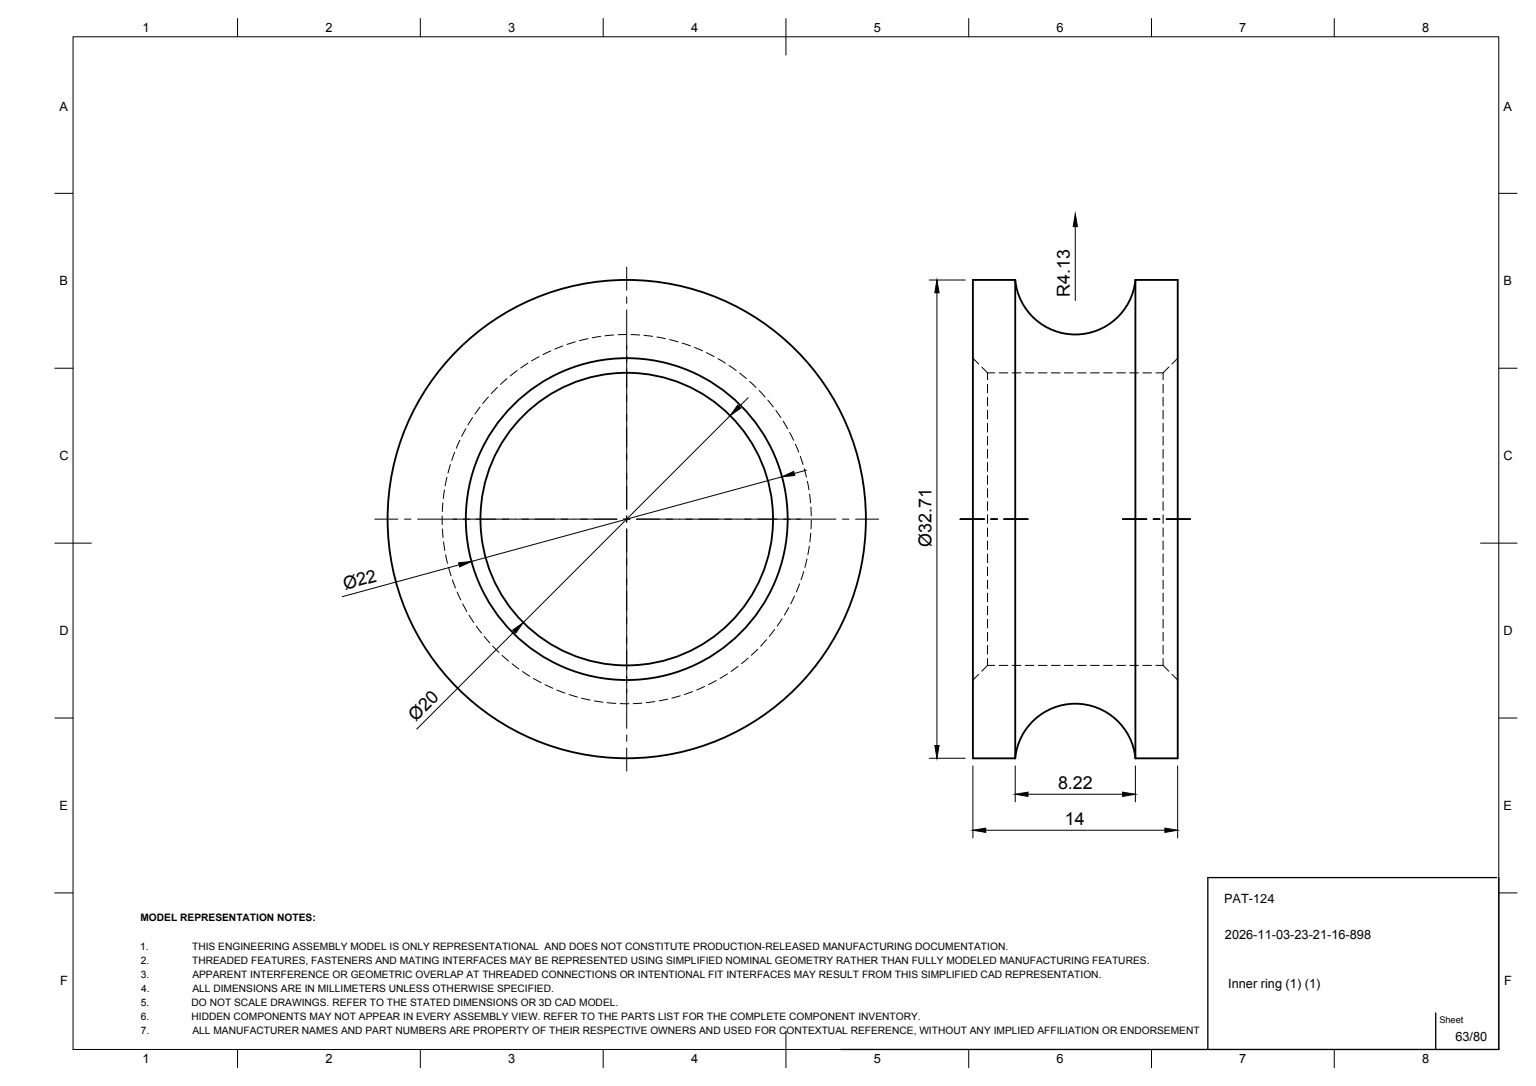
ISO-10303-21;
HEADER;
/* Generated by software containing ST-Developer
 * from STEP Tools, Inc. (www.steptools.com) 
 */

FILE_DESCRIPTION(
/* description */ ('XY cross-slide table'),
/* implementation_level */ '2;1');

FILE_NAME(
/* name */ 'Inner ring (1) (1).step',
/* time_stamp */ '2026-10-28T03:22:46-07:00',
/* author */ (''),
/* organization */ (''),
/* preprocessor_version */ 'ST-DEVELOPER v20.2',
/* originating_system */ 'Autodesk Translation Framework v15.17.0.0',
/* authorisation */ '');

FILE_SCHEMA (('AUTOMOTIVE_DESIGN { 1 0 10303 214 3 1 1 }'));
ENDSEC;

DATA;
#10=MECHANICAL_DESIGN_GEOMETRIC_PRESENTATION_REPRESENTATION('',(#1748),#62984);
#1471=CONICAL_SURFACE('',#25671,1.05,0.785398163397449);
#1472=CONICAL_SURFACE('',#25678,1.05,0.785398163397449);
#1502=TOROIDAL_SURFACE('',#25660,1.675,0.412776);
#1560=SHAPE_REPRESENTATION_RELATIONSHIP('SRR','None',#63417,#1643);
#1643=ADVANCED_BREP_SHAPE_REPRESENTATION('',(#1857),#62954);
#1748=STYLED_ITEM('',(#63912),#1857);
#1857=MANIFOLD_SOLID_BREP('Body1',#23046);
#2210=FACE_BOUND('',#5365,.T.);
#2211=FACE_BOUND('',#5368,.T.);
#2678=PLANE('',#25673);
#2679=PLANE('',#25676);
#3723=FACE_OUTER_BOUND('',#5360,.T.);
#3724=FACE_OUTER_BOUND('',#5361,.T.);
#3725=FACE_OUTER_BOUND('',#5362,.T.);
#3726=FACE_OUTER_BOUND('',#5363,.T.);
#3727=FACE_OUTER_BOUND('',#5364,.T.);
#3728=FACE_OUTER_BOUND('',#5366,.T.);
#3729=FACE_OUTER_BOUND('',#5367,.T.);
#3730=FACE_OUTER_BOUND('',#5369,.T.);
#5360=EDGE_LOOP('',(#18826,#18827,#18828,#18829,#18830,#18831));
#5361=EDGE_LOOP('',(#18832,#18833,#18834,#18835,#18836));
#5362=EDGE_LOOP('',(#18837,#18838,#18839,#18840));
#5363=EDGE_LOOP('',(#18841,#18842,#18843,#18844));
#5364=EDGE_LOOP('',(#18845));
#5365=EDGE_LOOP('',(#18846));
#5366=EDGE_LOOP('',(#18847,#18848,#18849,#18850,#18851));
#5367=EDGE_LOOP('',(#18852));
#5368=EDGE_LOOP('',(#18853));
#5369=EDGE_LOOP('',(#18854,#18855,#18856,#18857));
#6853=LINE('',#49072,#8340);
#6854=LINE('',#49078,#8341);
#6855=LINE('',#49082,#8342);
#6856=LINE('',#49088,#8343);
#6857=LINE('',#49093,#8344);
#8340=VECTOR('',#30742,1.63531);
#8341=VECTOR('',#30749,1.);
#8342=VECTOR('',#30754,1.05);
#8343=VECTOR('',#30763,1.63531);
#8344=VECTOR('',#30770,1.05);
#9536=CIRCLE('',#25661,1.63531);
#9537=CIRCLE('',#25662,1.63531);
#9538=CIRCLE('',#25663,0.412776);
#9539=CIRCLE('',#25664,1.63531);
#9540=CIRCLE('',#25665,1.63531);
#9541=CIRCLE('',#25667,1.63531);
#9542=CIRCLE('',#25669,1.);
#9543=CIRCLE('',#25670,1.);
#9544=CIRCLE('',#25672,1.1);
#9545=CIRCLE('',#25675,1.63531);
#9546=CIRCLE('',#25677,1.1);
#11095=VERTEX_POINT('',#49061);
#11096=VERTEX_POINT('',#49062);
#11097=VERTEX_POINT('',#49065);
#11098=VERTEX_POINT('',#49067);
#11099=VERTEX_POINT('',#49071);
#11100=VERTEX_POINT('',#49075);
#11101=VERTEX_POINT('',#49077);
#11102=VERTEX_POINT('',#49081);
#11103=VERTEX_POINT('',#49086);
#11104=VERTEX_POINT('',#49090);
#13797=EDGE_CURVE('',#11095,#11096,#9536,.T.);
#13798=EDGE_CURVE('',#11096,#11095,#9537,.T.);
#13799=EDGE_CURVE('',#11096,#11097,#9538,.T.);
#13800=EDGE_CURVE('',#11098,#11097,#9539,.T.);
#13801=EDGE_CURVE('',#11097,#11098,#9540,.T.);
#13802=EDGE_CURVE('',#11098,#11099,#6853,.T.);
#13803=EDGE_CURVE('',#11099,#11099,#9541,.T.);
#13804=EDGE_CURVE('',#11100,#11100,#9542,.T.);
#13805=EDGE_CURVE('',#11100,#11101,#6854,.T.);
#13806=EDGE_CURVE('',#11101,#11101,#9543,.T.);
#13807=EDGE_CURVE('',#11101,#11102,#6855,.T.);
#13808=EDGE_CURVE('',#11102,#11102,#9544,.T.);
#13809=EDGE_CURVE('',#11103,#11103,#9545,.T.);
#13810=EDGE_CURVE('',#11103,#11095,#6856,.T.);
#13811=EDGE_CURVE('',#11104,#11104,#9546,.T.);
#13812=EDGE_CURVE('',#11104,#11100,#6857,.T.);
#18826=ORIENTED_EDGE('',*,*,#13797,.F.);
#18827=ORIENTED_EDGE('',*,*,#13798,.F.);
#18828=ORIENTED_EDGE('',*,*,#13799,.T.);
#18829=ORIENTED_EDGE('',*,*,#13800,.F.);
#18830=ORIENTED_EDGE('',*,*,#13801,.F.);
#18831=ORIENTED_EDGE('',*,*,#13799,.F.);
#18832=ORIENTED_EDGE('',*,*,#13800,.T.);
#18833=ORIENTED_EDGE('',*,*,#13801,.T.);
#18834=ORIENTED_EDGE('',*,*,#13802,.T.);
#18835=ORIENTED_EDGE('',*,*,#13803,.T.);
#18836=ORIENTED_EDGE('',*,*,#13802,.F.);
#18837=ORIENTED_EDGE('',*,*,#13804,.T.);
#18838=ORIENTED_EDGE('',*,*,#13805,.T.);
#18839=ORIENTED_EDGE('',*,*,#13806,.F.);
#18840=ORIENTED_EDGE('',*,*,#13805,.F.);
#18841=ORIENTED_EDGE('',*,*,#13806,.T.);
#18842=ORIENTED_EDGE('',*,*,#13807,.T.);
#18843=ORIENTED_EDGE('',*,*,#13808,.F.);
#18844=ORIENTED_EDGE('',*,*,#13807,.F.);
#18845=ORIENTED_EDGE('',*,*,#13803,.F.);
#18846=ORIENTED_EDGE('',*,*,#13808,.T.);
#18847=ORIENTED_EDGE('',*,*,#13809,.F.);
#18848=ORIENTED_EDGE('',*,*,#13810,.T.);
#18849=ORIENTED_EDGE('',*,*,#13797,.T.);
#18850=ORIENTED_EDGE('',*,*,#13798,.T.);
#18851=ORIENTED_EDGE('',*,*,#13810,.F.);
#18852=ORIENTED_EDGE('',*,*,#13809,.T.);
#18853=ORIENTED_EDGE('',*,*,#13811,.F.);
#18854=ORIENTED_EDGE('',*,*,#13811,.T.);
#18855=ORIENTED_EDGE('',*,*,#13812,.T.);
#18856=ORIENTED_EDGE('',*,*,#13804,.F.);
#18857=ORIENTED_EDGE('',*,*,#13812,.F.);
#21428=CYLINDRICAL_SURFACE('',#25666,1.63531);
#21429=CYLINDRICAL_SURFACE('',#25668,1.);
#21430=CYLINDRICAL_SURFACE('',#25674,1.63531);
#22504=ADVANCED_FACE('',(#3723),#1502,.F.);
#22505=ADVANCED_FACE('',(#3724),#21428,.T.);
#22506=ADVANCED_FACE('',(#3725),#21429,.F.);
#22507=ADVANCED_FACE('',(#3726),#1471,.F.);
#22508=ADVANCED_FACE('',(#3727,#2210),#2678,.T.);
#22509=ADVANCED_FACE('',(#3728),#21430,.T.);
#22510=ADVANCED_FACE('',(#3729,#2211),#2679,.T.);
#22511=ADVANCED_FACE('',(#3730),#1472,.F.);
#23046=CLOSED_SHELL('',(#22504,#22505,#22506,#22507,#22508,#22509,#22510,
#22511));
#25659=AXIS2_PLACEMENT_3D('',#49059,#30726,#30727);
#25660=AXIS2_PLACEMENT_3D('',#49060,#30728,#30729);
#25661=AXIS2_PLACEMENT_3D('',#49063,#30730,#30731);
#25662=AXIS2_PLACEMENT_3D('',#49064,#30732,#30733);
#25663=AXIS2_PLACEMENT_3D('',#49066,#30734,#30735);
#25664=AXIS2_PLACEMENT_3D('',#49068,#30736,#30737);
#25665=AXIS2_PLACEMENT_3D('',#49069,#30738,#30739);
#25666=AXIS2_PLACEMENT_3D('',#49070,#30740,#30741);
#25667=AXIS2_PLACEMENT_3D('',#49073,#30743,#30744);
#25668=AXIS2_PLACEMENT_3D('',#49074,#30745,#30746);
#25669=AXIS2_PLACEMENT_3D('',#49076,#30747,#30748);
#25670=AXIS2_PLACEMENT_3D('',#49079,#30750,#30751);
#25671=AXIS2_PLACEMENT_3D('',#49080,#30752,#30753);
#25672=AXIS2_PLACEMENT_3D('',#49083,#30755,#30756);
#25673=AXIS2_PLACEMENT_3D('',#49084,#30757,#30758);
#25674=AXIS2_PLACEMENT_3D('',#49085,#30759,#30760);
#25675=AXIS2_PLACEMENT_3D('',#49087,#30761,#30762);
#25676=AXIS2_PLACEMENT_3D('',#49089,#30764,#30765);
#25677=AXIS2_PLACEMENT_3D('',#49091,#30766,#30767);
#25678=AXIS2_PLACEMENT_3D('',#49092,#30768,#30769);
#30726=DIRECTION('axis',(0.,0.,1.));
#30727=DIRECTION('refdir',(1.,0.,0.));
#30728=DIRECTION('center_axis',(0.,-1.,0.));
#30729=DIRECTION('ref_axis',(0.,0.,-1.));
#30730=DIRECTION('center_axis',(0.,-1.,0.));
#30731=DIRECTION('ref_axis',(1.,0.,0.));
#30732=DIRECTION('center_axis',(0.,-1.,0.));
#30733=DIRECTION('ref_axis',(1.,0.,0.));
#30734=DIRECTION('center_axis',(1.,0.,1.22464679914735E-16));
#30735=DIRECTION('ref_axis',(-1.22464679914735E-16,0.,1.));
#30736=DIRECTION('center_axis',(0.,1.,0.));
#30737=DIRECTION('ref_axis',(1.,0.,0.));
#30738=DIRECTION('center_axis',(0.,1.,0.));
#30739=DIRECTION('ref_axis',(1.,0.,0.));
#30740=DIRECTION('center_axis',(0.,-1.,0.));
#30741=DIRECTION('ref_axis',(1.,0.,0.));
#30742=DIRECTION('',(0.,1.,0.));
#30743=DIRECTION('center_axis',(0.,-1.,0.));
#30744=DIRECTION('ref_axis',(1.,0.,0.));
#30745=DIRECTION('center_axis',(0.,-1.,0.));
#30746=DIRECTION('ref_axis',(1.,0.,0.));
#30747=DIRECTION('center_axis',(0.,-1.,0.));
#30748=DIRECTION('ref_axis',(1.,0.,0.));
#30749=DIRECTION('',(0.,1.,0.));
#30750=DIRECTION('center_axis',(0.,-1.,0.));
#30751=DIRECTION('ref_axis',(1.,0.,0.));
#30752=DIRECTION('center_axis',(0.,1.,0.));
#30753=DIRECTION('ref_axis',(1.,0.,0.));
#30754=DIRECTION('',(-0.707106781186548,0.707106781186547,-8.65956056235494E-17));
#30755=DIRECTION('center_axis',(0.,-1.,0.));
#30756=DIRECTION('ref_axis',(1.,0.,0.));
#30757=DIRECTION('center_axis',(0.,1.,0.));
#30758=DIRECTION('ref_axis',(0.,0.,1.));
#30759=DIRECTION('center_axis',(0.,-1.,0.));
#30760=DIRECTION('ref_axis',(1.,0.,0.));
#30761=DIRECTION('center_axis',(0.,-1.,0.));
#30762=DIRECTION('ref_axis',(1.,0.,0.));
#30763=DIRECTION('',(0.,1.,0.));
#30764=DIRECTION('center_axis',(0.,-1.,0.));
#30765=DIRECTION('ref_axis',(0.,0.,-1.));
#30766=DIRECTION('center_axis',(0.,-1.,0.));
#30767=DIRECTION('ref_axis',(1.,0.,0.));
#30768=DIRECTION('center_axis',(0.,-1.,0.));
#30769=DIRECTION('ref_axis',(1.,0.,0.));
#30770=DIRECTION('',(0.707106781186548,0.707106781186547,8.65956056235494E-17));
#49059=CARTESIAN_POINT('',(0.,0.,0.));
#49060=CARTESIAN_POINT('Origin',(0.,0.,0.));
#49061=CARTESIAN_POINT('',(-1.63531,-0.410863395882378,-2.00267715711366E-16));
#49062=CARTESIAN_POINT('',(-2.00267715711366E-16,-0.410863395882378,1.63531));
#49063=CARTESIAN_POINT('Origin',(0.,-0.410863395882378,0.));
#49064=CARTESIAN_POINT('Origin',(0.,-0.410863395882378,0.));
#49065=CARTESIAN_POINT('',(-2.00267715711366E-16,0.410863395882378,1.63531));
#49066=CARTESIAN_POINT('Origin',(-2.05128338857182E-16,0.,1.675));
#49067=CARTESIAN_POINT('',(-1.63531,0.410863395882378,2.00267715711366E-16));
#49068=CARTESIAN_POINT('Origin',(0.,0.410863395882378,0.));
#49069=CARTESIAN_POINT('Origin',(0.,0.410863395882378,0.));
#49070=CARTESIAN_POINT('Origin',(0.,0.,0.));
#49071=CARTESIAN_POINT('',(-1.63531,0.7,-2.00267715711366E-16));
#49072=CARTESIAN_POINT('',(-1.63531,0.,-2.00267715711366E-16));
#49073=CARTESIAN_POINT('Origin',(0.,0.7,0.));
#49074=CARTESIAN_POINT('Origin',(0.,0.,0.));
#49075=CARTESIAN_POINT('',(-1.,-0.6,-1.22464679914735E-16));
#49076=CARTESIAN_POINT('Origin',(0.,-0.6,0.));
#49077=CARTESIAN_POINT('',(-1.,0.6,-1.22464679914735E-16));
#49078=CARTESIAN_POINT('',(-1.,0.,-1.22464679914735E-16));
#49079=CARTESIAN_POINT('Origin',(0.,0.6,0.));
#49080=CARTESIAN_POINT('Origin',(0.,0.65,0.));
#49081=CARTESIAN_POINT('',(-1.1,0.7,-1.34711147906209E-16));
#49082=CARTESIAN_POINT('',(-1.05,0.65,-1.28587913910472E-16));
#49083=CARTESIAN_POINT('Origin',(0.,0.7,0.));
#49084=CARTESIAN_POINT('Origin',(1.63531,0.7,0.));
#49085=CARTESIAN_POINT('Origin',(0.,0.,0.));
#49086=CARTESIAN_POINT('',(-1.63531,-0.7,-2.00267715711366E-16));
#49087=CARTESIAN_POINT('Origin',(0.,-0.7,0.));
#49088=CARTESIAN_POINT('',(-1.63531,0.,-2.00267715711366E-16));
#49089=CARTESIAN_POINT('Origin',(1.1,-0.7,0.));
#49090=CARTESIAN_POINT('',(-1.1,-0.7,-1.34711147906209E-16));
#49091=CARTESIAN_POINT('Origin',(0.,-0.7,0.));
#49092=CARTESIAN_POINT('Origin',(0.,-0.65,0.));
#49093=CARTESIAN_POINT('',(-1.05,-0.65,-1.28587913910472E-16));
#62855=UNCERTAINTY_MEASURE_WITH_UNIT(LENGTH_MEASURE(0.001),#62985,
'DISTANCE_ACCURACY_VALUE',
'Maximum model space distance between geometric entities at asserted c
onnectivities');
#62885=UNCERTAINTY_MEASURE_WITH_UNIT(LENGTH_MEASURE(0.001),#62985,
'DISTANCE_ACCURACY_VALUE',
'Maximum model space distance between geometric entities at asserted c
onnectivities');
#62954=(
GEOMETRIC_REPRESENTATION_CONTEXT(3)
GLOBAL_UNCERTAINTY_ASSIGNED_CONTEXT((#62855))
GLOBAL_UNIT_ASSIGNED_CONTEXT((#62985,#62987,#62988))
REPRESENTATION_CONTEXT('','3D')
);
#62984=(
GEOMETRIC_REPRESENTATION_CONTEXT(3)
GLOBAL_UNCERTAINTY_ASSIGNED_CONTEXT((#62885))
GLOBAL_UNIT_ASSIGNED_CONTEXT((#62985,#62987,#62988))
REPRESENTATION_CONTEXT('','3D')
);
#62985=(
LENGTH_UNIT()
NAMED_UNIT(*)
SI_UNIT(.CENTI.,.METRE.)
);
#62987=(
NAMED_UNIT(*)
PLANE_ANGLE_UNIT()
SI_UNIT($,.RADIAN.)
);
#62988=(
NAMED_UNIT(*)
SI_UNIT($,.STERADIAN.)
SOLID_ANGLE_UNIT()
);
#63057=SHAPE_DEFINITION_REPRESENTATION(#63240,#63417);
#63240=PRODUCT_DEFINITION_SHAPE('',$,#63516);
#63417=SHAPE_REPRESENTATION('',(#25659),#62954);
#63447=PRODUCT_DEFINITION_CONTEXT('part definition',#63743,'design');
#63516=PRODUCT_DEFINITION('Inner ring (1) (1)','Inner ring (1) (1)',#63614,
#63447);
#63614=PRODUCT_DEFINITION_FORMATION('',$,#63813);
#63743=APPLICATION_CONTEXT(
'Core Data for Automotive Mechanical Design Process');
#63744=PRODUCT_CONTEXT('part definition',#63743,'mechanical');
#63813=PRODUCT('Inner ring (1) (1)','Inner ring (1) (1)','Inner ring (1) (1)',(#63744));
#63906=COLOUR_RGB('Grey',0.48,0.52,0.57);
#63907=FILL_AREA_STYLE_COLOUR('',#63906);
#63908=FILL_AREA_STYLE('',(#63907));
#63909=SURFACE_STYLE_FILL_AREA(#63908);
#63910=SURFACE_SIDE_STYLE('',(#63909));
#63911=SURFACE_STYLE_USAGE(.BOTH.,#63910);
#63912=PRESENTATION_STYLE_ASSIGNMENT((#63911));
ENDSEC;
END-ISO-10303-21;
